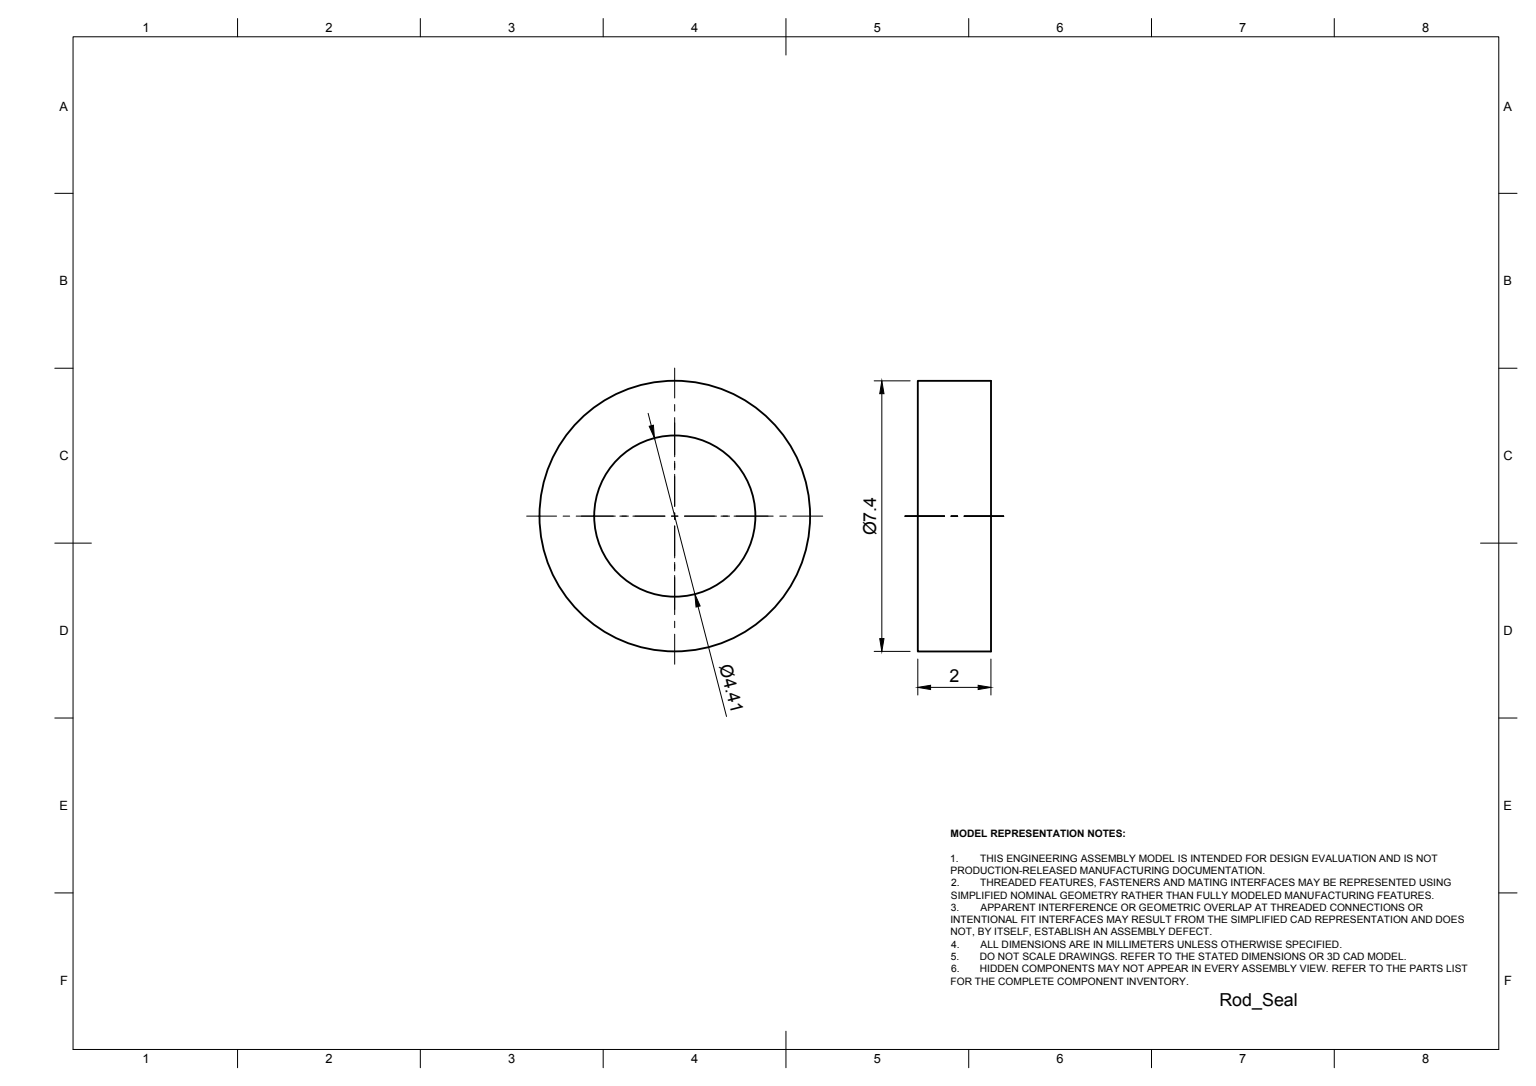
ISO-10303-21;
HEADER;
/* Generated by software containing ST-Developer
 * from STEP Tools, Inc. (www.steptools.com) 
 */

FILE_DESCRIPTION(
/* description */ (''),
/* implementation_level */ '2;1');

FILE_NAME(
/* name */ 'Rod_Seal.step',
/* time_stamp */ '2026-10-06T13:15:55-07:00',
/* author */ (''),
/* organization */ (''),
/* preprocessor_version */ 'ST-DEVELOPER v20.2',
/* originating_system */ 'Autodesk Translation Framework v15.15.0.0',
/* authorisation */ '');

FILE_SCHEMA (('AUTOMOTIVE_DESIGN { 1 0 10303 214 3 1 1 }'));
ENDSEC;

DATA;
#10=MECHANICAL_DESIGN_GEOMETRIC_PRESENTATION_REPRESENTATION('',(#117),#27707);
#97=SHAPE_REPRESENTATION_RELATIONSHIP('SRR','None',#27754,#107);
#107=ADVANCED_BREP_SHAPE_REPRESENTATION('',(#127),#27706);
#117=STYLED_ITEM('',(#27804),#127);
#127=MANIFOLD_SOLID_BREP('Body1',#3843);
#161=FACE_BOUND('',#911,.T.);
#162=FACE_BOUND('',#914,.T.);
#216=PLANE('',#4273);
#217=PLANE('',#4277);
#340=CIRCLE('',#4271,3.7);
#341=CIRCLE('',#4272,3.7);
#342=CIRCLE('',#4274,2.204);
#343=CIRCLE('',#4276,2.204);
#436=CYLINDRICAL_SURFACE('',#4270,3.7);
#437=CYLINDRICAL_SURFACE('',#4275,2.204);
#655=FACE_OUTER_BOUND('',#909,.T.);
#656=FACE_OUTER_BOUND('',#910,.T.);
#657=FACE_OUTER_BOUND('',#912,.T.);
#658=FACE_OUTER_BOUND('',#913,.T.);
#909=EDGE_LOOP('',(#3563,#3564,#3565,#3566));
#910=EDGE_LOOP('',(#3567));
#911=EDGE_LOOP('',(#3568));
#912=EDGE_LOOP('',(#3569,#3570,#3571,#3572));
#913=EDGE_LOOP('',(#3573));
#914=EDGE_LOOP('',(#3574));
#1089=LINE('',#27664,#1265);
#1090=LINE('',#27672,#1266);
#1265=VECTOR('',#5096,3.7);
#1266=VECTOR('',#5107,2.204);
#1894=VERTEX_POINT('',#27661);
#1895=VERTEX_POINT('',#27663);
#1896=VERTEX_POINT('',#27667);
#1897=VERTEX_POINT('',#27670);
#2451=EDGE_CURVE('',#1894,#1894,#340,.T.);
#2452=EDGE_CURVE('',#1894,#1895,#1089,.T.);
#2453=EDGE_CURVE('',#1895,#1895,#341,.T.);
#2454=EDGE_CURVE('',#1896,#1896,#342,.T.);
#2455=EDGE_CURVE('',#1897,#1897,#343,.T.);
#2456=EDGE_CURVE('',#1897,#1896,#1090,.T.);
#3563=ORIENTED_EDGE('',*,*,#2451,.F.);
#3564=ORIENTED_EDGE('',*,*,#2452,.T.);
#3565=ORIENTED_EDGE('',*,*,#2453,.T.);
#3566=ORIENTED_EDGE('',*,*,#2452,.F.);
#3567=ORIENTED_EDGE('',*,*,#2451,.T.);
#3568=ORIENTED_EDGE('',*,*,#2454,.F.);
#3569=ORIENTED_EDGE('',*,*,#2455,.F.);
#3570=ORIENTED_EDGE('',*,*,#2456,.T.);
#3571=ORIENTED_EDGE('',*,*,#2454,.T.);
#3572=ORIENTED_EDGE('',*,*,#2456,.F.);
#3573=ORIENTED_EDGE('',*,*,#2453,.F.);
#3574=ORIENTED_EDGE('',*,*,#2455,.T.);
#3830=ADVANCED_FACE('',(#655),#436,.T.);
#3831=ADVANCED_FACE('',(#656,#161),#216,.T.);
#3832=ADVANCED_FACE('',(#657),#437,.F.);
#3833=ADVANCED_FACE('',(#658,#162),#217,.T.);
#3843=CLOSED_SHELL('',(#3830,#3831,#3832,#3833));
#4269=AXIS2_PLACEMENT_3D('',#27659,#5090,#5091);
#4270=AXIS2_PLACEMENT_3D('',#27660,#5092,#5093);
#4271=AXIS2_PLACEMENT_3D('',#27662,#5094,#5095);
#4272=AXIS2_PLACEMENT_3D('',#27665,#5097,#5098);
#4273=AXIS2_PLACEMENT_3D('',#27666,#5099,#5100);
#4274=AXIS2_PLACEMENT_3D('',#27668,#5101,#5102);
#4275=AXIS2_PLACEMENT_3D('',#27669,#5103,#5104);
#4276=AXIS2_PLACEMENT_3D('',#27671,#5105,#5106);
#4277=AXIS2_PLACEMENT_3D('',#27673,#5108,#5109);
#5090=DIRECTION('axis',(0.,0.,1.));
#5091=DIRECTION('refdir',(1.,0.,0.));
#5092=DIRECTION('center_axis',(1.,0.,0.));
#5093=DIRECTION('ref_axis',(0.,1.,0.));
#5094=DIRECTION('center_axis',(1.,0.,0.));
#5095=DIRECTION('ref_axis',(0.,0.,-1.));
#5096=DIRECTION('',(-1.,0.,0.));
#5097=DIRECTION('center_axis',(1.,0.,0.));
#5098=DIRECTION('ref_axis',(0.,0.,-1.));
#5099=DIRECTION('center_axis',(1.,0.,0.));
#5100=DIRECTION('ref_axis',(0.,0.,-1.));
#5101=DIRECTION('center_axis',(1.,0.,0.));
#5102=DIRECTION('ref_axis',(0.,0.,-1.));
#5103=DIRECTION('center_axis',(1.,0.,0.));
#5104=DIRECTION('ref_axis',(0.,1.,0.));
#5105=DIRECTION('center_axis',(1.,0.,0.));
#5106=DIRECTION('ref_axis',(0.,0.,-1.));
#5107=DIRECTION('',(1.,0.,0.));
#5108=DIRECTION('center_axis',(-1.,0.,0.));
#5109=DIRECTION('ref_axis',(0.,0.,1.));
#27659=CARTESIAN_POINT('',(0.,0.,0.));
#27660=CARTESIAN_POINT('Origin',(80.44,0.,0.));
#27661=CARTESIAN_POINT('',(81.44,-3.7,-4.53119315684521E-16));
#27662=CARTESIAN_POINT('Origin',(81.44,0.,0.));
#27663=CARTESIAN_POINT('',(79.44,-3.7,-4.53119315684521E-16));
#27664=CARTESIAN_POINT('',(80.44,-3.7,-4.53119315684521E-16));
#27665=CARTESIAN_POINT('Origin',(79.44,0.,0.));
#27666=CARTESIAN_POINT('Origin',(81.44,2.204,0.));
#27667=CARTESIAN_POINT('',(81.44,-2.204,-2.69912154532077E-16));
#27668=CARTESIAN_POINT('Origin',(81.44,0.,0.));
#27669=CARTESIAN_POINT('Origin',(80.44,0.,0.));
#27670=CARTESIAN_POINT('',(79.44,-2.204,-2.69912154532077E-16));
#27671=CARTESIAN_POINT('Origin',(79.44,0.,0.));
#27672=CARTESIAN_POINT('',(80.44,-2.204,-2.69912154532077E-16));
#27673=CARTESIAN_POINT('Origin',(79.44,3.7,0.));
#27694=UNCERTAINTY_MEASURE_WITH_UNIT(LENGTH_MEASURE(0.01),#27708,
'DISTANCE_ACCURACY_VALUE',
'Maximum model space distance between geometric entities at asserted c
onnectivities');
#27695=UNCERTAINTY_MEASURE_WITH_UNIT(LENGTH_MEASURE(0.01),#27708,
'DISTANCE_ACCURACY_VALUE',
'Maximum model space distance between geometric entities at asserted c
onnectivities');
#27706=(
GEOMETRIC_REPRESENTATION_CONTEXT(3)
GLOBAL_UNCERTAINTY_ASSIGNED_CONTEXT((#27694))
GLOBAL_UNIT_ASSIGNED_CONTEXT((#27708,#27710,#27711))
REPRESENTATION_CONTEXT('','3D')
);
#27707=(
GEOMETRIC_REPRESENTATION_CONTEXT(3)
GLOBAL_UNCERTAINTY_ASSIGNED_CONTEXT((#27695))
GLOBAL_UNIT_ASSIGNED_CONTEXT((#27708,#27710,#27711))
REPRESENTATION_CONTEXT('','3D')
);
#27708=(
LENGTH_UNIT()
NAMED_UNIT(*)
SI_UNIT(.MILLI.,.METRE.)
);
#27710=(
NAMED_UNIT(*)
PLANE_ANGLE_UNIT()
SI_UNIT($,.RADIAN.)
);
#27711=(
NAMED_UNIT(*)
SI_UNIT($,.STERADIAN.)
SOLID_ANGLE_UNIT()
);
#27722=SHAPE_DEFINITION_REPRESENTATION(#27733,#27754);
#27733=PRODUCT_DEFINITION_SHAPE('',$,#27766);
#27754=SHAPE_REPRESENTATION('',(#4269),#27706);
#27755=PRODUCT_DEFINITION_CONTEXT('part definition',#27790,'design');
#27766=PRODUCT_DEFINITION('2026-10-01-22-51-42-851','Rod_Seal',#27777,#27755);
#27777=PRODUCT_DEFINITION_FORMATION('',$,#27802);
#27790=APPLICATION_CONTEXT(
'Core Data for Automotive Mechanical Design Process');
#27791=PRODUCT_CONTEXT('part definition',#27790,'mechanical');
#27802=PRODUCT('2026-10-01-22-51-42-851','Rod_Seal',$,(#27791));
#27804=PRESENTATION_STYLE_ASSIGNMENT((#27806));
#27806=SURFACE_STYLE_USAGE(.BOTH.,#27808);
#27808=SURFACE_SIDE_STYLE('',(#27810));
#27810=SURFACE_STYLE_FILL_AREA(#27812);
#27812=FILL_AREA_STYLE('Opaque(160,160,160)',(#27814));
#27814=FILL_AREA_STYLE_COLOUR('Opaque(160,160,160)',#27816);
#27816=COLOUR_RGB('Opaque(160,160,160)', 0.09019608, 0.27058824, 0.51372549);
ENDSEC;
END-ISO-10303-21;
